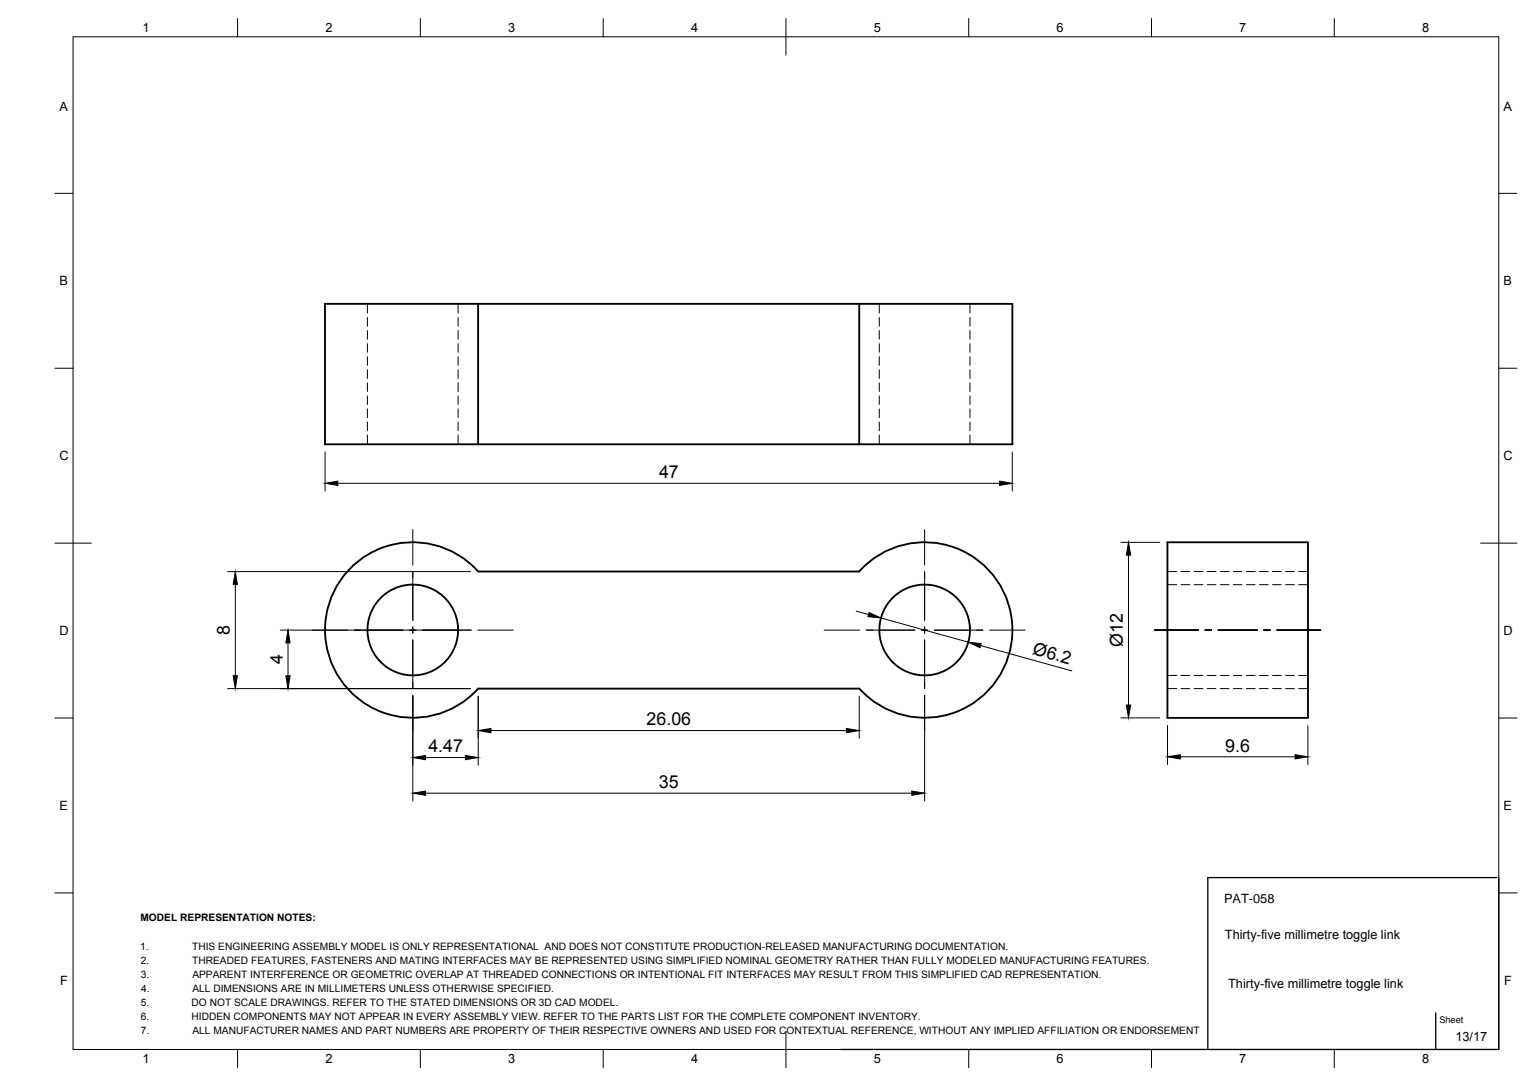
ISO-10303-21;
HEADER;
/* Generated by software containing ST-Developer
 * from STEP Tools, Inc. (www.steptools.com) 
 */

FILE_DESCRIPTION(
/* description */ ('Horizontal push-pull toggle clamp'),
/* implementation_level */ '2;1');

FILE_NAME(
/* name */ 'Thirty-five millimetre toggle link.step',
/* time_stamp */ '2026-10-27T21:21:09-07:00',
/* author */ (''),
/* organization */ (''),
/* preprocessor_version */ 'ST-DEVELOPER v20.2',
/* originating_system */ 'Autodesk Translation Framework v15.17.0.0',
/* authorisation */ '');

FILE_SCHEMA (('AUTOMOTIVE_DESIGN { 1 0 10303 214 3 1 1 }'));
ENDSEC;

DATA;
#10=MECHANICAL_DESIGN_GEOMETRIC_PRESENTATION_REPRESENTATION('',(#189),#4791);
#163=SHAPE_REPRESENTATION_RELATIONSHIP('SRR','None',#4868,#176);
#176=ADVANCED_BREP_SHAPE_REPRESENTATION('',(#201),#4781);
#189=STYLED_ITEM('',(#5037),#201);
#201=MANIFOLD_SOLID_BREP('Body1',#2634);
#236=FACE_BOUND('',#624,.T.);
#237=FACE_BOUND('',#625,.T.);
#238=FACE_BOUND('',#629,.T.);
#239=FACE_BOUND('',#630,.T.);
#317=PLANE('',#2926);
#318=PLANE('',#2927);
#319=PLANE('',#2929);
#320=PLANE('',#2932);
#442=FACE_OUTER_BOUND('',#619,.T.);
#443=FACE_OUTER_BOUND('',#620,.T.);
#444=FACE_OUTER_BOUND('',#621,.T.);
#445=FACE_OUTER_BOUND('',#622,.T.);
#446=FACE_OUTER_BOUND('',#623,.T.);
#447=FACE_OUTER_BOUND('',#626,.T.);
#448=FACE_OUTER_BOUND('',#627,.T.);
#449=FACE_OUTER_BOUND('',#628,.T.);
#619=EDGE_LOOP('',(#2149,#2150,#2151,#2152));
#620=EDGE_LOOP('',(#2153,#2154,#2155,#2156));
#621=EDGE_LOOP('',(#2157,#2158,#2159,#2160));
#622=EDGE_LOOP('',(#2161,#2162,#2163,#2164));
#623=EDGE_LOOP('',(#2165,#2166,#2167,#2168));
#624=EDGE_LOOP('',(#2169));
#625=EDGE_LOOP('',(#2170));
#626=EDGE_LOOP('',(#2171,#2172,#2173,#2174));
#627=EDGE_LOOP('',(#2175,#2176,#2177,#2178));
#628=EDGE_LOOP('',(#2179,#2180,#2181,#2182));
#629=EDGE_LOOP('',(#2183));
#630=EDGE_LOOP('',(#2184));
#751=CIRCLE('',#2918,0.31);
#752=CIRCLE('',#2919,0.31);
#753=CIRCLE('',#2921,0.31);
#754=CIRCLE('',#2922,0.31);
#755=CIRCLE('',#2924,0.6);
#756=CIRCLE('',#2925,0.6);
#757=CIRCLE('',#2928,0.6);
#758=CIRCLE('',#2931,0.6);
#938=LINE('',#4253,#1158);
#939=LINE('',#4259,#1159);
#940=LINE('',#4264,#1160);
#941=LINE('',#4268,#1161);
#942=LINE('',#4272,#1162);
#943=LINE('',#4274,#1163);
#944=LINE('',#4275,#1164);
#945=LINE('',#4278,#1165);
#946=LINE('',#4282,#1166);
#947=LINE('',#4283,#1167);
#1158=VECTOR('',#3476,0.31);
#1159=VECTOR('',#3483,0.31);
#1160=VECTOR('',#3488,1.);
#1161=VECTOR('',#3491,1.);
#1162=VECTOR('',#3496,1.);
#1163=VECTOR('',#3497,1.);
#1164=VECTOR('',#3498,1.);
#1165=VECTOR('',#3501,1.);
#1166=VECTOR('',#3506,1.);
#1167=VECTOR('',#3507,1.);
#1357=VERTEX_POINT('',#4250);
#1358=VERTEX_POINT('',#4252);
#1359=VERTEX_POINT('',#4256);
#1360=VERTEX_POINT('',#4258);
#1361=VERTEX_POINT('',#4262);
#1362=VERTEX_POINT('',#4263);
#1363=VERTEX_POINT('',#4265);
#1364=VERTEX_POINT('',#4267);
#1365=VERTEX_POINT('',#4271);
#1366=VERTEX_POINT('',#4273);
#1367=VERTEX_POINT('',#4277);
#1368=VERTEX_POINT('',#4281);
#1636=EDGE_CURVE('',#1357,#1357,#751,.T.);
#1637=EDGE_CURVE('',#1357,#1358,#938,.T.);
#1638=EDGE_CURVE('',#1358,#1358,#752,.T.);
#1639=EDGE_CURVE('',#1359,#1359,#753,.T.);
#1640=EDGE_CURVE('',#1359,#1360,#939,.T.);
#1641=EDGE_CURVE('',#1360,#1360,#754,.T.);
#1642=EDGE_CURVE('',#1361,#1362,#940,.T.);
#1643=EDGE_CURVE('',#1363,#1361,#755,.T.);
#1644=EDGE_CURVE('',#1364,#1363,#941,.T.);
#1645=EDGE_CURVE('',#1364,#1362,#756,.T.);
#1646=EDGE_CURVE('',#1362,#1365,#942,.T.);
#1647=EDGE_CURVE('',#1366,#1365,#943,.T.);
#1648=EDGE_CURVE('',#1361,#1366,#944,.T.);
#1649=EDGE_CURVE('',#1367,#1364,#945,.T.);
#1650=EDGE_CURVE('',#1365,#1367,#757,.T.);
#1651=EDGE_CURVE('',#1368,#1363,#946,.T.);
#1652=EDGE_CURVE('',#1367,#1368,#947,.T.);
#1653=EDGE_CURVE('',#1366,#1368,#758,.T.);
#2149=ORIENTED_EDGE('',*,*,#1636,.F.);
#2150=ORIENTED_EDGE('',*,*,#1637,.T.);
#2151=ORIENTED_EDGE('',*,*,#1638,.F.);
#2152=ORIENTED_EDGE('',*,*,#1637,.F.);
#2153=ORIENTED_EDGE('',*,*,#1639,.F.);
#2154=ORIENTED_EDGE('',*,*,#1640,.T.);
#2155=ORIENTED_EDGE('',*,*,#1641,.F.);
#2156=ORIENTED_EDGE('',*,*,#1640,.F.);
#2157=ORIENTED_EDGE('',*,*,#1642,.F.);
#2158=ORIENTED_EDGE('',*,*,#1643,.F.);
#2159=ORIENTED_EDGE('',*,*,#1644,.F.);
#2160=ORIENTED_EDGE('',*,*,#1645,.T.);
#2161=ORIENTED_EDGE('',*,*,#1642,.T.);
#2162=ORIENTED_EDGE('',*,*,#1646,.T.);
#2163=ORIENTED_EDGE('',*,*,#1647,.F.);
#2164=ORIENTED_EDGE('',*,*,#1648,.F.);
#2165=ORIENTED_EDGE('',*,*,#1645,.F.);
#2166=ORIENTED_EDGE('',*,*,#1649,.F.);
#2167=ORIENTED_EDGE('',*,*,#1650,.F.);
#2168=ORIENTED_EDGE('',*,*,#1646,.F.);
#2169=ORIENTED_EDGE('',*,*,#1636,.T.);
#2170=ORIENTED_EDGE('',*,*,#1639,.T.);
#2171=ORIENTED_EDGE('',*,*,#1644,.T.);
#2172=ORIENTED_EDGE('',*,*,#1651,.F.);
#2173=ORIENTED_EDGE('',*,*,#1652,.F.);
#2174=ORIENTED_EDGE('',*,*,#1649,.T.);
#2175=ORIENTED_EDGE('',*,*,#1647,.T.);
#2176=ORIENTED_EDGE('',*,*,#1650,.T.);
#2177=ORIENTED_EDGE('',*,*,#1652,.T.);
#2178=ORIENTED_EDGE('',*,*,#1653,.F.);
#2179=ORIENTED_EDGE('',*,*,#1648,.T.);
#2180=ORIENTED_EDGE('',*,*,#1653,.T.);
#2181=ORIENTED_EDGE('',*,*,#1651,.T.);
#2182=ORIENTED_EDGE('',*,*,#1643,.T.);
#2183=ORIENTED_EDGE('',*,*,#1638,.T.);
#2184=ORIENTED_EDGE('',*,*,#1641,.T.);
#2459=CYLINDRICAL_SURFACE('',#2917,0.31);
#2460=CYLINDRICAL_SURFACE('',#2920,0.31);
#2461=CYLINDRICAL_SURFACE('',#2923,0.6);
#2462=CYLINDRICAL_SURFACE('',#2930,0.6);
#2558=ADVANCED_FACE('',(#442),#2459,.F.);
#2559=ADVANCED_FACE('',(#443),#2460,.F.);
#2560=ADVANCED_FACE('',(#444),#2461,.T.);
#2561=ADVANCED_FACE('',(#445),#317,.T.);
#2562=ADVANCED_FACE('',(#446,#236,#237),#318,.F.);
#2563=ADVANCED_FACE('',(#447),#319,.T.);
#2564=ADVANCED_FACE('',(#448),#2462,.T.);
#2565=ADVANCED_FACE('',(#449,#238,#239),#320,.T.);
#2634=CLOSED_SHELL('',(#2558,#2559,#2560,#2561,#2562,#2563,#2564,#2565));
#2916=AXIS2_PLACEMENT_3D('',#4248,#3470,#3471);
#2917=AXIS2_PLACEMENT_3D('',#4249,#3472,#3473);
#2918=AXIS2_PLACEMENT_3D('',#4251,#3474,#3475);
#2919=AXIS2_PLACEMENT_3D('',#4254,#3477,#3478);
#2920=AXIS2_PLACEMENT_3D('',#4255,#3479,#3480);
#2921=AXIS2_PLACEMENT_3D('',#4257,#3481,#3482);
#2922=AXIS2_PLACEMENT_3D('',#4260,#3484,#3485);
#2923=AXIS2_PLACEMENT_3D('',#4261,#3486,#3487);
#2924=AXIS2_PLACEMENT_3D('',#4266,#3489,#3490);
#2925=AXIS2_PLACEMENT_3D('',#4269,#3492,#3493);
#2926=AXIS2_PLACEMENT_3D('',#4270,#3494,#3495);
#2927=AXIS2_PLACEMENT_3D('',#4276,#3499,#3500);
#2928=AXIS2_PLACEMENT_3D('',#4279,#3502,#3503);
#2929=AXIS2_PLACEMENT_3D('',#4280,#3504,#3505);
#2930=AXIS2_PLACEMENT_3D('',#4284,#3508,#3509);
#2931=AXIS2_PLACEMENT_3D('',#4285,#3510,#3511);
#2932=AXIS2_PLACEMENT_3D('',#4286,#3512,#3513);
#3470=DIRECTION('axis',(0.,0.,1.));
#3471=DIRECTION('refdir',(1.,0.,0.));
#3472=DIRECTION('center_axis',(0.,1.,0.));
#3473=DIRECTION('ref_axis',(1.,0.,0.));
#3474=DIRECTION('center_axis',(0.,1.,0.));
#3475=DIRECTION('ref_axis',(1.,0.,0.));
#3476=DIRECTION('',(0.,1.,0.));
#3477=DIRECTION('center_axis',(0.,-1.,0.));
#3478=DIRECTION('ref_axis',(1.,0.,0.));
#3479=DIRECTION('center_axis',(0.,1.,0.));
#3480=DIRECTION('ref_axis',(1.,0.,0.));
#3481=DIRECTION('center_axis',(0.,1.,0.));
#3482=DIRECTION('ref_axis',(1.,0.,0.));
#3483=DIRECTION('',(0.,1.,0.));
#3484=DIRECTION('center_axis',(0.,-1.,0.));
#3485=DIRECTION('ref_axis',(1.,0.,0.));
#3486=DIRECTION('center_axis',(0.,1.,0.));
#3487=DIRECTION('ref_axis',(1.,0.,0.));
#3488=DIRECTION('',(0.,-1.,0.));
#3489=DIRECTION('center_axis',(0.,1.,0.));
#3490=DIRECTION('ref_axis',(1.,0.,0.));
#3491=DIRECTION('',(0.,1.,0.));
#3492=DIRECTION('center_axis',(0.,1.,0.));
#3493=DIRECTION('ref_axis',(1.,0.,0.));
#3494=DIRECTION('center_axis',(0.062254101962613,0.,-0.998060332238903));
#3495=DIRECTION('ref_axis',(-0.998060332238903,0.,-0.062254101962613));
#3496=DIRECTION('',(-0.998060332238903,0.,-0.062254101962613));
#3497=DIRECTION('',(0.,-1.,0.));
#3498=DIRECTION('',(-0.998060332238903,0.,-0.062254101962613));
#3499=DIRECTION('center_axis',(0.,1.,0.));
#3500=DIRECTION('ref_axis',(1.,0.,0.));
#3501=DIRECTION('',(0.998060332238903,0.,0.062254101962613));
#3502=DIRECTION('center_axis',(0.,1.,0.));
#3503=DIRECTION('ref_axis',(1.,0.,0.));
#3504=DIRECTION('center_axis',(-0.062254101962613,0.,0.998060332238903));
#3505=DIRECTION('ref_axis',(0.998060332238903,0.,0.062254101962613));
#3506=DIRECTION('',(0.998060332238903,0.,0.062254101962613));
#3507=DIRECTION('',(0.,1.,0.));
#3508=DIRECTION('center_axis',(0.,1.,0.));
#3509=DIRECTION('ref_axis',(-0.998060332238903,0.,-0.0622541019626133));
#3510=DIRECTION('center_axis',(0.,1.,0.));
#3511=DIRECTION('ref_axis',(1.,0.,0.));
#3512=DIRECTION('center_axis',(0.,1.,0.));
#3513=DIRECTION('ref_axis',(1.,0.,0.));
#4248=CARTESIAN_POINT('',(0.,0.,0.));
#4249=CARTESIAN_POINT('Origin',(2.49048674522936,-0.6,2.28211064313085));
#4250=CARTESIAN_POINT('',(2.18048674522936,-0.48,2.28211064313085));
#4251=CARTESIAN_POINT('Origin',(2.49048674522936,-0.48,2.28211064313085));
#4252=CARTESIAN_POINT('',(2.18048674522936,0.48,2.28211064313085));
#4253=CARTESIAN_POINT('',(2.18048674522936,-0.6,2.28211064313085));
#4254=CARTESIAN_POINT('Origin',(2.49048674522936,0.48,2.28211064313085));
#4255=CARTESIAN_POINT('Origin',(5.98369790806552,-0.6,2.5));
#4256=CARTESIAN_POINT('',(5.67369790806552,-0.48,2.5));
#4257=CARTESIAN_POINT('Origin',(5.98369790806552,-0.48,2.5));
#4258=CARTESIAN_POINT('',(5.67369790806552,0.48,2.5));
#4259=CARTESIAN_POINT('',(5.67369790806552,-0.6,2.5));
#4260=CARTESIAN_POINT('Origin',(5.98369790806552,0.48,2.5));
#4261=CARTESIAN_POINT('Origin',(5.98369790806552,-0.48,2.5));
#4262=CARTESIAN_POINT('',(5.56225339914413,0.48,2.07293498633112));
#4263=CARTESIAN_POINT('',(5.56225339914413,-0.48,2.07293498633112));
#4264=CARTESIAN_POINT('',(5.56225339914413,-0.48,2.07293498633112));
#4265=CARTESIAN_POINT('',(5.51245011757404,0.48,2.87138325212224));
#4266=CARTESIAN_POINT('Origin',(5.98369790806552,0.48,2.5));
#4267=CARTESIAN_POINT('',(5.51245011757404,-0.48,2.87138325212224));
#4268=CARTESIAN_POINT('',(5.51245011757404,-0.48,2.87138325212224));
#4269=CARTESIAN_POINT('Origin',(5.98369790806552,-0.48,2.5));
#4270=CARTESIAN_POINT('Origin',(6.00859954885057,-0.48,2.10077586710444));
#4271=CARTESIAN_POINT('',(2.96173453572085,-0.48,1.91072739100861));
#4272=CARTESIAN_POINT('',(6.00859954885057,-0.48,2.10077586710444));
#4273=CARTESIAN_POINT('',(2.96173453572085,0.48,1.91072739100861));
#4274=CARTESIAN_POINT('',(2.96173453572085,-0.48,1.91072739100861));
#4275=CARTESIAN_POINT('',(6.00859954885057,0.48,2.10077586710444));
#4276=CARTESIAN_POINT('Origin',(2.49048674522936,-0.48,2.28211064313085));
#4277=CARTESIAN_POINT('',(2.91193125415076,-0.48,2.70917565679974));
#4278=CARTESIAN_POINT('',(2.46558510444432,-0.48,2.68133477602642));
#4279=CARTESIAN_POINT('Origin',(2.49048674522936,-0.48,2.28211064313085));
#4280=CARTESIAN_POINT('Origin',(2.46558510444432,-0.48,2.68133477602642));
#4281=CARTESIAN_POINT('',(2.91193125415076,0.48,2.70917565679974));
#4282=CARTESIAN_POINT('',(2.46558510444432,0.48,2.68133477602642));
#4283=CARTESIAN_POINT('',(2.91193125415076,-0.48,2.70917565679974));
#4284=CARTESIAN_POINT('Origin',(2.49048674522936,-0.48,2.28211064313085));
#4285=CARTESIAN_POINT('Origin',(2.49048674522936,0.48,2.28211064313085));
#4286=CARTESIAN_POINT('Origin',(2.49048674522936,0.48,2.28211064313085));
#4762=UNCERTAINTY_MEASURE_WITH_UNIT(LENGTH_MEASURE(0.001),#4792,
'DISTANCE_ACCURACY_VALUE',
'Maximum model space distance between geometric entities at asserted c
onnectivities');
#4772=UNCERTAINTY_MEASURE_WITH_UNIT(LENGTH_MEASURE(0.001),#4792,
'DISTANCE_ACCURACY_VALUE',
'Maximum model space distance between geometric entities at asserted c
onnectivities');
#4781=(
GEOMETRIC_REPRESENTATION_CONTEXT(3)
GLOBAL_UNCERTAINTY_ASSIGNED_CONTEXT((#4762))
GLOBAL_UNIT_ASSIGNED_CONTEXT((#4792,#4794,#4795))
REPRESENTATION_CONTEXT('','3D')
);
#4791=(
GEOMETRIC_REPRESENTATION_CONTEXT(3)
GLOBAL_UNCERTAINTY_ASSIGNED_CONTEXT((#4772))
GLOBAL_UNIT_ASSIGNED_CONTEXT((#4792,#4794,#4795))
REPRESENTATION_CONTEXT('','3D')
);
#4792=(
LENGTH_UNIT()
NAMED_UNIT(*)
SI_UNIT(.CENTI.,.METRE.)
);
#4794=(
NAMED_UNIT(*)
PLANE_ANGLE_UNIT()
SI_UNIT($,.RADIAN.)
);
#4795=(
NAMED_UNIT(*)
SI_UNIT($,.STERADIAN.)
SOLID_ANGLE_UNIT()
);
#4804=SHAPE_DEFINITION_REPRESENTATION(#4822,#4868);
#4822=PRODUCT_DEFINITION_SHAPE('',$,#4887);
#4868=SHAPE_REPRESENTATION('',(#2916),#4781);
#4878=PRODUCT_DEFINITION_CONTEXT('part definition',#4934,'design');
#4887=PRODUCT_DEFINITION('Thirty-five millimetre toggle link',
'Thirty-five millimetre toggle link',#4905,#4878);
#4905=PRODUCT_DEFINITION_FORMATION('',$,#4944);
#4934=APPLICATION_CONTEXT(
'Core Data for Automotive Mechanical Design Process');
#4935=PRODUCT_CONTEXT('part definition',#4934,'mechanical');
#4944=PRODUCT('Thirty-five millimetre toggle link',
'Thirty-five millimetre toggle link',
'Thirty-five millimetre toggle link',(#4935));
#5031=COLOUR_RGB('Off White',0.89,0.88,0.83);
#5032=FILL_AREA_STYLE_COLOUR('',#5031);
#5033=FILL_AREA_STYLE('',(#5032));
#5034=SURFACE_STYLE_FILL_AREA(#5033);
#5035=SURFACE_SIDE_STYLE('',(#5034));
#5036=SURFACE_STYLE_USAGE(.BOTH.,#5035);
#5037=PRESENTATION_STYLE_ASSIGNMENT((#5036));
ENDSEC;
END-ISO-10303-21;
